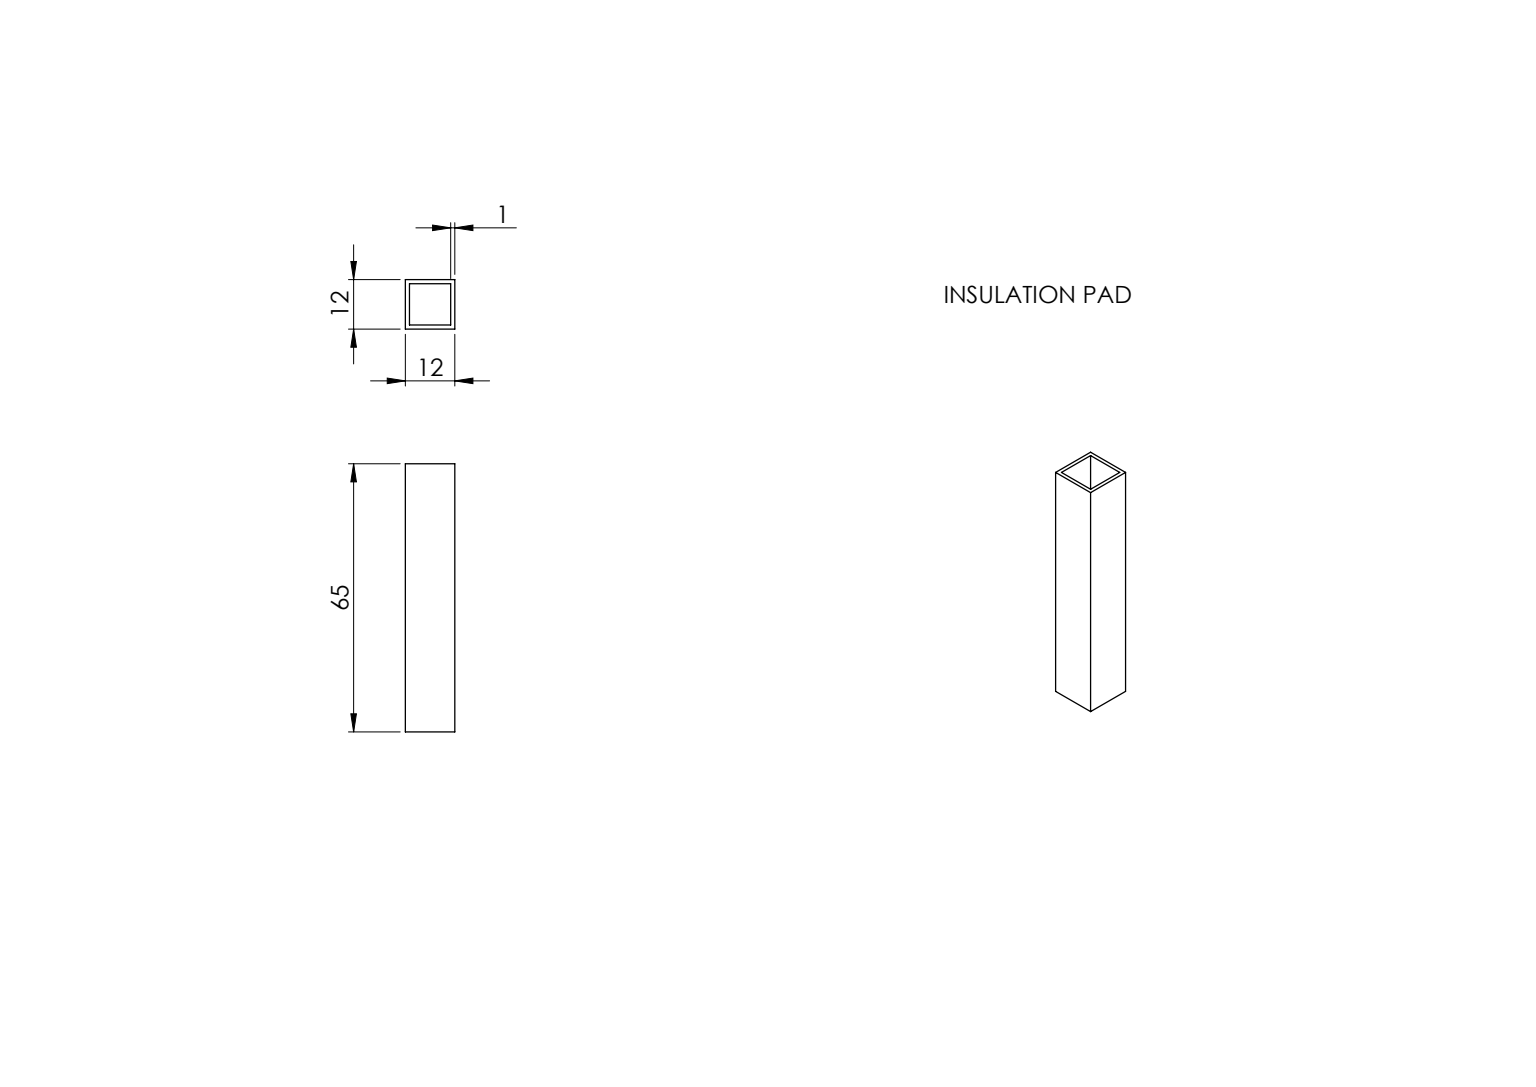
ISO-10303-21;
HEADER;
FILE_DESCRIPTION (('STEP AP214'),
    '1' );
FILE_NAME ('Insulation Pad.step',
    '2026-10-24T04:45:50',
    ( '' ),
    ( '' ),
    'SwSTEP 2.0',
    'SolidWorks 2026',
    '' );
FILE_SCHEMA (( 'AUTOMOTIVE_DESIGN' ));
ENDSEC;

DATA;
#9=LINE ( 'NONE', #3109, #1942 ) ;
#10=ORIENTED_EDGE ( 'NONE', *, *, #1397, .T. ) ;
#12=FILL_AREA_STYLE_COLOUR ( '', #2947 ) ;
#16=EDGE_CURVE ( 'NONE', #2394, #756, #2740, .T. ) ;
#20=CARTESIAN_POINT ( 'NONE',  ( -40.00000000000000000, 136.9705627484771355, -4.999999999999995559 ) ) ;
#23=CARTESIAN_POINT ( 'NONE',  ( -49.99999999999999289, 136.9705627484771355, -4.999999999999995559 ) ) ;
#29=LINE ( 'NONE', #1074, #3100 ) ;
#37=PLANE ( 'NONE',  #2989 ) ;
#53=CARTESIAN_POINT ( 'NONE',  ( -51.00000000000000000, 52.00000000000000711, -5.999999999999995559 ) ) ;
#60=EDGE_CURVE ( 'NONE', #1345, #1406, #445, .T. ) ;
#63=SHAPE_REPRESENTATION_RELATIONSHIP ( 'NONE' , 'NONE' ,  #2804, #1506 ) ;
#67=LINE ( 'NONE', #1330, #689 ) ;
#83=CARTESIAN_POINT ( 'NONE',  ( -51.00000000000000711, 136.9705627484771355, 6.000000000000004441 ) ) ;
#84=VERTEX_POINT ( 'NONE', #2233 ) ;
#102=EDGE_LOOP ( 'NONE', ( #2901, #2851, #579, #3094 ) ) ;
#105=PLANE ( 'NONE',  #1846 ) ;
#108=VERTEX_POINT ( 'NONE', #676 ) ;
#120=ORIENTED_EDGE ( 'NONE', *, *, #698, .T. ) ;
#127=ORIENTED_EDGE ( 'NONE', *, *, #1397, .F. ) ;
#136=CARTESIAN_POINT ( 'NONE',  ( 0.000000000000000000, 117.0000000000000000, 0.000000000000000000 ) ) ;
#152=VECTOR ( 'NONE', #2701, 1000.000000000000000 ) ;
#156=DIRECTION ( 'NONE',  ( 1.000000000000000000, 0.000000000000000000, -0.000000000000000000 ) ) ;
#161=MECHANICAL_DESIGN_GEOMETRIC_PRESENTATION_REPRESENTATION('',(#2503),#1797);
#164=VECTOR ( 'NONE', #3281, 1000.000000000000000 ) ;
#196=CARTESIAN_POINT ( 'NONE',  ( -51.00000000000000000, 136.9705627484771355, -5.999999999999995559 ) ) ;
#215=CARTESIAN_POINT ( 'NONE',  ( -40.00000000000000000, 52.00000000000000711, -4.999999999999995559 ) ) ;
#237=EDGE_LOOP ( 'NONE', ( #1273, #3223, #1162, #2040 ) ) ;
#241=EDGE_CURVE ( 'NONE', #1406, #684, #9, .T. ) ;
#253=CARTESIAN_POINT ( 'NONE',  ( -40.00000000000000000, 52.00000000000000711, 5.000000000000004441 ) ) ;
#265=DIRECTION ( 'NONE',  ( 0.000000000000000000, 0.000000000000000000, -1.000000000000000000 ) ) ;
#278=ORIENTED_EDGE ( 'NONE', *, *, #1945, .T. ) ;
#280=DIRECTION ( 'NONE',  ( 0.000000000000000000, 0.000000000000000000, -1.000000000000000000 ) ) ;
#305=LINE ( 'NONE', #901, #2667 ) ;
#309=VERTEX_POINT ( 'NONE', #1378 ) ;
#339=LINE ( 'NONE', #83, #1798 ) ;
#357=FACE_BOUND ( 'NONE', #1452, .T. ) ;
#380=DIRECTION ( 'NONE',  ( 0.000000000000000000, -0.000000000000000000, 1.000000000000000000 ) ) ;
#394=DIRECTION ( 'NONE',  ( 0.000000000000000000, 0.000000000000000000, 1.000000000000000000 ) ) ;
#406=CARTESIAN_POINT ( 'NONE',  ( -51.00000000000000000, 136.9705627484771355, -4.999999999999996447 ) ) ;
#409=EDGE_CURVE ( 'NONE', #2129, #108, #67, .T. ) ;
#412=PLANE ( 'NONE',  #1407 ) ;
#418=LINE ( 'NONE', #2471, #152 ) ;
#419=CARTESIAN_POINT ( 'NONE',  ( -50.00000000000000000, 117.0000000000000000, 5.000000000000004441 ) ) ;
#442=PLANE ( 'NONE',  #2112 ) ;
#445=LINE ( 'NONE', #3298, #1076 ) ;
#451=EDGE_LOOP ( 'NONE', ( #1435, #993, #1013, #2138 ) ) ;
#459=EDGE_CURVE ( 'NONE', #756, #1406, #418, .T. ) ;
#475=DIRECTION ( 'NONE',  ( 0.000000000000000000, -1.000000000000000000, 0.000000000000000000 ) ) ;
#490=CARTESIAN_POINT ( 'NONE',  ( -39.00000000000000000, 52.00000000000000711, -5.999999999999995559 ) ) ;
#505=SURFACE_SIDE_STYLE ('',( #2583 ) ) ;
#509=LINE ( 'NONE', #2809, #1520 ) ;
#540=VECTOR ( 'NONE', #639, 1000.000000000000000 ) ;
#568=ORIENTED_EDGE ( 'NONE', *, *, #3327, .T. ) ;
#578=PLANE ( 'NONE',  #2006 ) ;
#579=ORIENTED_EDGE ( 'NONE', *, *, #3144, .T. ) ;
#612=DIRECTION ( 'NONE',  ( 0.000000000000000000, 0.000000000000000000, 1.000000000000000000 ) ) ;
#625=VERTEX_POINT ( 'NONE', #215 ) ;
#627=CARTESIAN_POINT ( 'NONE',  ( -40.00000000000000000, 136.9705627484771355, -5.999999999999995559 ) ) ;
#632=ORIENTED_EDGE ( 'NONE', *, *, #2958, .F. ) ;
#634=LINE ( 'NONE', #948, #2276 ) ;
#639=DIRECTION ( 'NONE',  ( 1.000000000000000000, 0.000000000000000000, 0.000000000000000000 ) ) ;
#641=AXIS2_PLACEMENT_3D ( 'NONE', #1222, #3272, #3009 ) ;
#647=DIRECTION ( 'NONE',  ( -0.000000000000000000, -1.000000000000000000, -0.000000000000000000 ) ) ;
#649=VECTOR ( 'NONE', #3280, 1000.000000000000000 ) ;
#664=CARTESIAN_POINT ( 'NONE',  ( -49.99999999999999289, 136.9705627484771355, -4.999999999999995559 ) ) ;
#676=CARTESIAN_POINT ( 'NONE',  ( -40.00000000000000000, 117.0000000000000000, 5.000000000000004441 ) ) ;
#684=VERTEX_POINT ( 'NONE', #490 ) ;
#689=VECTOR ( 'NONE', #1588, 1000.000000000000000 ) ;
#698=EDGE_CURVE ( 'NONE', #2833, #625, #1646, .T. ) ;
#705=ORIENTED_EDGE ( 'NONE', *, *, #2348, .T. ) ;
#713=CARTESIAN_POINT ( 'NONE',  ( -50.00000000000000000, 117.0000000000000000, 5.000000000000004441 ) ) ;
#716=DIRECTION ( 'NONE',  ( -0.000000000000000000, -1.000000000000000000, -0.000000000000000000 ) ) ;
#718=ORIENTED_EDGE ( 'NONE', *, *, #60, .T. ) ;
#726=EDGE_LOOP ( 'NONE', ( #2242, #1959, #3250, #1072 ) ) ;
#729=DIRECTION ( 'NONE',  ( -1.000000000000000000, 0.000000000000000000, 0.000000000000000000 ) ) ;
#734=FACE_OUTER_BOUND ( 'NONE', #1714, .T. ) ;
#746=CARTESIAN_POINT ( 'NONE',  ( -39.00000000000000000, 136.9705627484771355, 5.000000000000004441 ) ) ;
#747=( LENGTH_UNIT ( ) NAMED_UNIT ( * ) SI_UNIT ( .MILLI., .METRE. ) );
#756=VERTEX_POINT ( 'NONE', #1175 ) ;
#761=VECTOR ( 'NONE', #1874, 1000.000000000000000 ) ;
#780=ORIENTED_EDGE ( 'NONE', *, *, #1489, .F. ) ;
#790=CARTESIAN_POINT ( 'NONE',  ( -50.00000000000000000, 136.9705627484771355, 5.000000000000004441 ) ) ;
#833=CARTESIAN_POINT ( 'NONE',  ( -39.00000000000000000, 136.9705627484771355, -5.999999999999995559 ) ) ;
#839=ORIENTED_EDGE ( 'NONE', *, *, #241, .T. ) ;
#854=FACE_OUTER_BOUND ( 'NONE', #1573, .T. ) ;
#868=EDGE_CURVE ( 'NONE', #2623, #2345, #2510, .T. ) ;
#879=ADVANCED_FACE ( 'NONE', ( #3023 ), #2238, .T. ) ;
#901=CARTESIAN_POINT ( 'NONE',  ( -49.99999999999999289, 117.0000000000000000, -4.999999999999995559 ) ) ;
#924=CARTESIAN_POINT ( 'NONE',  ( -50.00000000000000000, 136.9705627484771355, 6.000000000000004441 ) ) ;
#943=ORIENTED_EDGE ( 'NONE', *, *, #459, .F. ) ;
#948=CARTESIAN_POINT ( 'NONE',  ( -50.00000000000000000, 136.9705627484771355, 5.000000000000004441 ) ) ;
#955=DIRECTION ( 'NONE',  ( 1.000000000000000000, 0.000000000000000000, 0.000000000000000000 ) ) ;
#960=ADVANCED_FACE ( 'NONE', ( #734 ), #412, .T. ) ;
#967=LINE ( 'NONE', #419, #649 ) ;
#985=STYLED_ITEM ( 'NONE', ( #3121 ), #1506 ) ;
#987=EDGE_LOOP ( 'NONE', ( #2562, #705, #1656, #127 ) ) ;
#993=ORIENTED_EDGE ( 'NONE', *, *, #16, .F. ) ;
#995=DIRECTION ( 'NONE',  ( 0.000000000000000000, -0.000000000000000000, 1.000000000000000000 ) ) ;
#1013=ORIENTED_EDGE ( 'NONE', *, *, #1945, .F. ) ;
#1016=EDGE_LOOP ( 'NONE', ( #943, #568, #1889, #718 ) ) ;
#1021=EDGE_CURVE ( 'NONE', #84, #309, #1844, .T. ) ;
#1043=ADVANCED_FACE ( 'NONE', ( #2321 ), #2375, .T. ) ;
#1048=ORIENTED_EDGE ( 'NONE', *, *, #3063, .F. ) ;
#1052=ADVANCED_FACE ( 'NONE', ( #1083 ), #37, .T. ) ;
#1072=ORIENTED_EDGE ( 'NONE', *, *, #1390, .F. ) ;
#1074=CARTESIAN_POINT ( 'NONE',  ( -40.00000000000000000, 52.00000000000000711, -5.999999999999995559 ) ) ;
#1076=VECTOR ( 'NONE', #955, 1000.000000000000000 ) ;
#1083=FACE_OUTER_BOUND ( 'NONE', #237, .T. ) ;
#1102=LINE ( 'NONE', #3195, #761 ) ;
#1112=( NAMED_UNIT ( * ) SI_UNIT ( $, .STERADIAN. ) SOLID_ANGLE_UNIT ( ) );
#1132=DIRECTION ( 'NONE',  ( -0.000000000000000000, -1.000000000000000000, -0.000000000000000000 ) ) ;
#1162=ORIENTED_EDGE ( 'NONE', *, *, #1845, .F. ) ;
#1175=CARTESIAN_POINT ( 'NONE',  ( -39.00000000000000000, 117.0000000000000000, 6.000000000000004441 ) ) ;
#1193=CARTESIAN_POINT ( 'NONE',  ( -40.00000000000000000, 117.0000000000000000, -5.999999999999995559 ) ) ;
#1200=DIRECTION ( 'NONE',  ( -1.000000000000000000, 0.000000000000000000, -0.000000000000000000 ) ) ;
#1221=ORIENTED_EDGE ( 'NONE', *, *, #868, .T. ) ;
#1222=CARTESIAN_POINT ( 'NONE',  ( -40.00000000000000000, 136.9705627484771355, 5.000000000000004441 ) ) ;
#1232=DIRECTION ( 'NONE',  ( 0.000000000000000000, 0.000000000000000000, -1.000000000000000000 ) ) ;
#1263=( GEOMETRIC_REPRESENTATION_CONTEXT ( 3 ) GLOBAL_UNCERTAINTY_ASSIGNED_CONTEXT ( ( #2493 ) ) GLOBAL_UNIT_ASSIGNED_CONTEXT ( ( #1560, #1854, #1112 ) ) REPRESENTATION_CONTEXT ( 'NONE', 'WORKASPACE' ) );
#1273=ORIENTED_EDGE ( 'NONE', *, *, #1950, .F. ) ;
#1292=ORIENTED_EDGE ( 'NONE', *, *, #241, .F. ) ;
#1311=EDGE_CURVE ( 'NONE', #625, #2623, #2265, .T. ) ;
#1330=CARTESIAN_POINT ( 'NONE',  ( -40.00000000000000000, 117.0000000000000000, 5.000000000000004441 ) ) ;
#1334=ORIENTED_EDGE ( 'NONE', *, *, #3070, .T. ) ;
#1341=ADVANCED_FACE ( 'NONE', ( #3314 ), #2522, .F. ) ;
#1345=VERTEX_POINT ( 'NONE', #1961 ) ;
#1370=DIRECTION ( 'NONE',  ( 0.000000000000000000, 1.000000000000000000, -0.000000000000000000 ) ) ;
#1378=CARTESIAN_POINT ( 'NONE',  ( -51.00000000000000000, 117.0000000000000000, -5.999999999999995559 ) ) ;
#1382=ORIENTED_EDGE ( 'NONE', *, *, #1311, .F. ) ;
#1389=EDGE_LOOP ( 'NONE', ( #1221, #2124, #120, #3042 ) ) ;
#1390=EDGE_CURVE ( 'NONE', #108, #2833, #3056, .T. ) ;
#1397=EDGE_CURVE ( 'NONE', #3137, #2623, #1940, .T. ) ;
#1406=VERTEX_POINT ( 'NONE', #2234 ) ;
#1407=AXIS2_PLACEMENT_3D ( 'NONE', #3287, #995, #156 ) ;
#1435=ORIENTED_EDGE ( 'NONE', *, *, #3327, .F. ) ;
#1452=EDGE_LOOP ( 'NONE', ( #1334, #2743, #2444, #3065 ) ) ;
#1460=DIRECTION ( 'NONE',  ( 6.938893903907229364E-16, 0.000000000000000000, -1.000000000000000000 ) ) ;
#1484=CARTESIAN_POINT ( 'NONE',  ( -40.00000000000000000, 52.00000000000000711, -4.999999999999995559 ) ) ;
#1489=EDGE_CURVE ( 'NONE', #3137, #2129, #509, .T. ) ;
#1506=ADVANCED_BREP_SHAPE_REPRESENTATION ( '', ( #2945, #3111 ), #2889 ) ;
#1520=VECTOR ( 'NONE', #3073, 1000.000000000000000 ) ;
#1522=EDGE_LOOP ( 'NONE', ( #632, #2728, #1292, #2496 ) ) ;
#1526=PRODUCT_DEFINITION ( 'UNKNOWN', '', #2020, #3077 ) ;
#1540=DIRECTION ( 'NONE',  ( 1.000000000000000000, -0.000000000000000000, 6.938893903907229364E-16 ) ) ;
#1552=( NAMED_UNIT ( * ) SI_UNIT ( $, .STERADIAN. ) SOLID_ANGLE_UNIT ( ) );
#1560=( LENGTH_UNIT ( ) NAMED_UNIT ( * ) SI_UNIT ( .MILLI., .METRE. ) );
#1573=EDGE_LOOP ( 'NONE', ( #2660, #278, #1578, #1896 ) ) ;
#1574=DIRECTION ( 'NONE',  ( 6.938893903907229364E-16, 0.000000000000000000, -1.000000000000000000 ) ) ;
#1578=ORIENTED_EDGE ( 'NONE', *, *, #3063, .T. ) ;
#1588=DIRECTION ( 'NONE',  ( 0.000000000000000000, 0.000000000000000000, 1.000000000000000000 ) ) ;
#1602=DIRECTION ( 'NONE',  ( 0.000000000000000000, 0.000000000000000000, 1.000000000000000000 ) ) ;
#1616=ADVANCED_FACE ( 'NONE', ( #3086 ), #2849, .F. ) ;
#1646=LINE ( 'NONE', #2175, #2002 ) ;
#1649=CARTESIAN_POINT ( 'NONE',  ( -40.00000000000000000, 117.0000000000000000, -4.999999999999995559 ) ) ;
#1656=ORIENTED_EDGE ( 'NONE', *, *, #868, .F. ) ;
#1679=ORIENTED_EDGE ( 'NONE', *, *, #16, .T. ) ;
#1682=AXIS2_PLACEMENT_3D ( 'NONE', #23, #1540, #1574 ) ;
#1693=CARTESIAN_POINT ( 'NONE',  ( -39.00000000000000000, 117.0000000000000000, 5.000000000000004441 ) ) ;
#1711=UNCERTAINTY_MEASURE_WITH_UNIT (LENGTH_MEASURE( 1.000000000000000082E-05 ), #3067, 'distance_accuracy_value', 'NONE');
#1714=EDGE_LOOP ( 'NONE', ( #780, #10, #1382, #3341 ) ) ;
#1785=CARTESIAN_POINT ( 'NONE',  ( -50.00000000000000000, 117.0000000000000000, 6.000000000000004441 ) ) ;
#1793=VECTOR ( 'NONE', #716, 1000.000000000000000 ) ;
#1796=CARTESIAN_POINT ( 'NONE',  ( -51.00000000000000000, 117.0000000000000000, -4.999999999999996447 ) ) ;
#1797=( GEOMETRIC_REPRESENTATION_CONTEXT ( 3 ) GLOBAL_UNCERTAINTY_ASSIGNED_CONTEXT ( ( #2842 ) ) GLOBAL_UNIT_ASSIGNED_CONTEXT ( ( #747, #2575, #1552 ) ) REPRESENTATION_CONTEXT ( 'NONE', 'WORKASPACE' ) );
#1798=VECTOR ( 'NONE', #1132, 1000.000000000000000 ) ;
#1815=ADVANCED_FACE ( 'NONE', ( #1973 ), #442, .F. ) ;
#1825=DIRECTION ( 'NONE',  ( 6.938893903907229364E-16, 0.000000000000000000, -1.000000000000000000 ) ) ;
#1829=( NAMED_UNIT ( * ) SI_UNIT ( $, .STERADIAN. ) SOLID_ANGLE_UNIT ( ) );
#1833=LINE ( 'NONE', #1785, #2288 ) ;
#1844=LINE ( 'NONE', #1796, #2336 ) ;
#1845=EDGE_CURVE ( 'NONE', #2345, #2833, #2245, .T. ) ;
#1846=AXIS2_PLACEMENT_3D ( 'NONE', #136, #475, #2537 ) ;
#1854=( NAMED_UNIT ( * ) PLANE_ANGLE_UNIT ( ) SI_UNIT ( $, .RADIAN. ) );
#1871=CARTESIAN_POINT ( 'NONE',  ( 0.000000000000000000, 0.000000000000000000, 0.000000000000000000 ) ) ;
#1874=DIRECTION ( 'NONE',  ( -6.938893903907228378E-16, 0.000000000000000000, 1.000000000000000000 ) ) ;
#1879=DIRECTION ( 'NONE',  ( 1.000000000000000000, 0.000000000000000000, -0.000000000000000000 ) ) ;
#1889=ORIENTED_EDGE ( 'NONE', *, *, #3125, .T. ) ;
#1896=ORIENTED_EDGE ( 'NONE', *, *, #2101, .T. ) ;
#1916=CARTESIAN_POINT ( 'NONE',  ( -49.99999999999999289, 52.00000000000000711, -4.999999999999995559 ) ) ;
#1930=PLANE ( 'NONE',  #2497 ) ;
#1940=LINE ( 'NONE', #664, #3326 ) ;
#1942=VECTOR ( 'NONE', #2794, 1000.000000000000000 ) ;
#1945=EDGE_CURVE ( 'NONE', #309, #2394, #3248, .T. ) ;
#1950=EDGE_CURVE ( 'NONE', #108, #3133, #967, .T. ) ;
#1959=ORIENTED_EDGE ( 'NONE', *, *, #2868, .T. ) ;
#1961=CARTESIAN_POINT ( 'NONE',  ( -51.00000000000000711, 52.00000000000000711, 6.000000000000004441 ) ) ;
#1967=PRODUCT_CONTEXT ( 'NONE', #2725, 'mechanical' ) ;
#1973=FACE_OUTER_BOUND ( 'NONE', #102, .T. ) ;
#2002=VECTOR ( 'NONE', #265, 1000.000000000000000 ) ;
#2006=AXIS2_PLACEMENT_3D ( 'NONE', #2957, #1370, #612 ) ;
#2020=PRODUCT_DEFINITION_FORMATION_WITH_SPECIFIED_SOURCE ( 'ANY', '', #2551, .NOT_KNOWN. ) ;
#2039=PRODUCT_DEFINITION_SHAPE ( 'NONE', 'NONE',  #1526 ) ;
#2040=ORIENTED_EDGE ( 'NONE', *, *, #2348, .F. ) ;
#2101=EDGE_CURVE ( 'NONE', #684, #3122, #29, .T. ) ;
#2105=CLOSED_SHELL ( 'NONE', ( #2661, #1815, #1341, #1616, #2638, #1043, #1052, #879, #960, #2738 ) ) ;
#2112=AXIS2_PLACEMENT_3D ( 'NONE', #406, #2979, #1460 ) ;
#2124=ORIENTED_EDGE ( 'NONE', *, *, #1845, .T. ) ;
#2129=VERTEX_POINT ( 'NONE', #1649 ) ;
#2130=MECHANICAL_DESIGN_GEOMETRIC_PRESENTATION_REPRESENTATION('',(#985),#1263);
#2138=ORIENTED_EDGE ( 'NONE', *, *, #1021, .F. ) ;
#2175=CARTESIAN_POINT ( 'NONE',  ( -40.00000000000000000, 52.00000000000000711, 5.000000000000004441 ) ) ;
#2200=DIRECTION ( 'NONE',  ( -0.000000000000000000, -1.000000000000000000, -0.000000000000000000 ) ) ;
#2210=CARTESIAN_POINT ( 'NONE',  ( -50.00000000000000000, 52.00000000000000711, 5.000000000000004441 ) ) ;
#2215=CARTESIAN_POINT ( 'NONE',  ( -40.00000000000000000, 136.9705627484771355, 5.000000000000004441 ) ) ;
#2233=CARTESIAN_POINT ( 'NONE',  ( -51.00000000000000711, 117.0000000000000000, 6.000000000000004441 ) ) ;
#2234=CARTESIAN_POINT ( 'NONE',  ( -39.00000000000000000, 52.00000000000000711, 6.000000000000004441 ) ) ;
#2238=PLANE ( 'NONE',  #641 ) ;
#2242=ORIENTED_EDGE ( 'NONE', *, *, #409, .F. ) ;
#2245=LINE ( 'NONE', #3030, #540 ) ;
#2247=CARTESIAN_POINT ( 'NONE',  ( -49.99999999999999289, 117.0000000000000000, -4.999999999999995559 ) ) ;
#2265=LINE ( 'NONE', #1484, #2281 ) ;
#2276=VECTOR ( 'NONE', #2719, 1000.000000000000000 ) ;
#2281=VECTOR ( 'NONE', #2506, 1000.000000000000000 ) ;
#2288=VECTOR ( 'NONE', #729, 1000.000000000000000 ) ;
#2296=( NAMED_UNIT ( * ) PLANE_ANGLE_UNIT ( ) SI_UNIT ( $, .RADIAN. ) );
#2321=FACE_OUTER_BOUND ( 'NONE', #987, .T. ) ;
#2326=SURFACE_STYLE_USAGE ( .BOTH. , #505 ) ;
#2336=VECTOR ( 'NONE', #1825, 1000.000000000000000 ) ;
#2345=VERTEX_POINT ( 'NONE', #2210 ) ;
#2348=EDGE_CURVE ( 'NONE', #3133, #2345, #634, .T. ) ;
#2375=PLANE ( 'NONE',  #1682 ) ;
#2384=AXIS2_PLACEMENT_3D ( 'NONE', #746, #2589, #1602 ) ;
#2394=VERTEX_POINT ( 'NONE', #3119 ) ;
#2418=LINE ( 'NONE', #833, #2556 ) ;
#2441=FACE_OUTER_BOUND ( 'NONE', #451, .T. ) ;
#2444=ORIENTED_EDGE ( 'NONE', *, *, #409, .T. ) ;
#2447=AXIS2_PLACEMENT_3D ( 'NONE', #924, #1232, #1200 ) ;
#2463=FACE_OUTER_BOUND ( 'NONE', #1522, .T. ) ;
#2471=CARTESIAN_POINT ( 'NONE',  ( -39.00000000000000000, 136.9705627484771355, 6.000000000000004441 ) ) ;
#2486=LINE ( 'NONE', #196, #164 ) ;
#2493=UNCERTAINTY_MEASURE_WITH_UNIT (LENGTH_MEASURE( 1.000000000000000082E-05 ), #1560, 'distance_accuracy_value', 'NONE');
#2496=ORIENTED_EDGE ( 'NONE', *, *, #60, .F. ) ;
#2497=AXIS2_PLACEMENT_3D ( 'NONE', #627, #380, #1879 ) ;
#2503=STYLED_ITEM('',(#3408),#2945);
#2506=DIRECTION ( 'NONE',  ( -1.000000000000000000, 0.000000000000000000, 0.000000000000000000 ) ) ;
#2510=LINE ( 'NONE', #2733, #2659 ) ;
#2522=PLANE ( 'NONE',  #2447 ) ;
#2537=DIRECTION ( 'NONE',  ( 0.000000000000000000, -0.000000000000000000, -1.000000000000000000 ) ) ;
#2551=PRODUCT ( 'Insulation Pad', 'Insulation Pad', '', ( #1967 ) ) ;
#2556=VECTOR ( 'NONE', #2200, 1000.000000000000000 ) ;
#2561=LINE ( 'NONE', #20, #2884 ) ;
#2562=ORIENTED_EDGE ( 'NONE', *, *, #3070, .F. ) ;
#2575=( NAMED_UNIT ( * ) PLANE_ANGLE_UNIT ( ) SI_UNIT ( $, .RADIAN. ) );
#2583=SURFACE_STYLE_FILL_AREA ( #2821 ) ;
#2589=DIRECTION ( 'NONE',  ( -1.000000000000000000, 0.000000000000000000, 0.000000000000000000 ) ) ;
#2612=DIRECTION ( 'NONE',  ( -0.000000000000000000, -1.000000000000000000, -0.000000000000000000 ) ) ;
#2623=VERTEX_POINT ( 'NONE', #1916 ) ;
#2638=ADVANCED_FACE ( 'NONE', ( #854 ), #1930, .F. ) ;
#2639=DIRECTION ( 'NONE',  ( 1.000000000000000000, 0.000000000000000000, 0.000000000000000000 ) ) ;
#2659=VECTOR ( 'NONE', #3062, 1000.000000000000000 ) ;
#2660=ORIENTED_EDGE ( 'NONE', *, *, #3144, .F. ) ;
#2661=ADVANCED_FACE ( 'NONE', ( #2463, #3253 ), #578, .F. ) ;
#2667=VECTOR ( 'NONE', #2982, 1000.000000000000000 ) ;
#2672=DIRECTION ( 'NONE',  ( -1.000000000000000000, 0.000000000000000000, 0.000000000000000000 ) ) ;
#2701=DIRECTION ( 'NONE',  ( -0.000000000000000000, -1.000000000000000000, -0.000000000000000000 ) ) ;
#2719=DIRECTION ( 'NONE',  ( -0.000000000000000000, -1.000000000000000000, -0.000000000000000000 ) ) ;
#2725=APPLICATION_CONTEXT ( 'automotive_design' ) ;
#2728=ORIENTED_EDGE ( 'NONE', *, *, #2101, .F. ) ;
#2733=CARTESIAN_POINT ( 'NONE',  ( -49.99999999999999289, 52.00000000000000711, -4.999999999999995559 ) ) ;
#2738=ADVANCED_FACE ( 'NONE', ( #357, #2441 ), #105, .F. ) ;
#2740=LINE ( 'NONE', #1693, #3087 ) ;
#2743=ORIENTED_EDGE ( 'NONE', *, *, #1489, .T. ) ;
#2794=DIRECTION ( 'NONE',  ( 0.000000000000000000, 0.000000000000000000, -1.000000000000000000 ) ) ;
#2804=SHAPE_REPRESENTATION ( 'Insulation Pad', ( #3111 ), #2889 ) ;
#2809=CARTESIAN_POINT ( 'NONE',  ( -40.00000000000000000, 117.0000000000000000, -4.999999999999995559 ) ) ;
#2821=FILL_AREA_STYLE ('',( #12 ) ) ;
#2833=VERTEX_POINT ( 'NONE', #253 ) ;
#2842=UNCERTAINTY_MEASURE_WITH_UNIT (LENGTH_MEASURE( 1.000000000000000082E-05 ), #747, 'distance_accuracy_value', 'NONE');
#2849=PLANE ( 'NONE',  #2384 ) ;
#2851=ORIENTED_EDGE ( 'NONE', *, *, #1021, .T. ) ;
#2868=EDGE_CURVE ( 'NONE', #2129, #625, #2561, .T. ) ;
#2872=VECTOR ( 'NONE', #3310, 1000.000000000000000 ) ;
#2884=VECTOR ( 'NONE', #2612, 1000.000000000000000 ) ;
#2889=( GEOMETRIC_REPRESENTATION_CONTEXT ( 3 ) GLOBAL_UNCERTAINTY_ASSIGNED_CONTEXT ( ( #1711 ) ) GLOBAL_UNIT_ASSIGNED_CONTEXT ( ( #3067, #2296, #1829 ) ) REPRESENTATION_CONTEXT ( 'NONE', 'WORKASPACE' ) );
#2900=APPLICATION_CONTEXT ( 'automotive_design' ) ;
#2901=ORIENTED_EDGE ( 'NONE', *, *, #3125, .F. ) ;
#2945=MANIFOLD_SOLID_BREP ( 'Extrude-Thin1', #2105 ) ;
#2947=COLOUR_RGB ( '',0.8941176470588234615, 0.8941176470588234615, 0.8941176470588234615 ) ;
#2957=CARTESIAN_POINT ( 'NONE',  ( 0.000000000000000000, 52.00000000000000711, 0.000000000000000000 ) ) ;
#2958=EDGE_CURVE ( 'NONE', #3122, #1345, #1102, .T. ) ;
#2979=DIRECTION ( 'NONE',  ( 1.000000000000000000, -0.000000000000000000, 6.938893903907229364E-16 ) ) ;
#2982=DIRECTION ( 'NONE',  ( 6.938893903907229364E-16, 0.000000000000000000, -1.000000000000000000 ) ) ;
#2989=AXIS2_PLACEMENT_3D ( 'NONE', #790, #280, #3170 ) ;
#3009=DIRECTION ( 'NONE',  ( 0.000000000000000000, 0.000000000000000000, 1.000000000000000000 ) ) ;
#3023=FACE_OUTER_BOUND ( 'NONE', #726, .T. ) ;
#3030=CARTESIAN_POINT ( 'NONE',  ( -50.00000000000000000, 52.00000000000000711, 5.000000000000004441 ) ) ;
#3042=ORIENTED_EDGE ( 'NONE', *, *, #1311, .T. ) ;
#3056=LINE ( 'NONE', #2215, #1793 ) ;
#3062=DIRECTION ( 'NONE',  ( -6.938893903907228378E-16, 0.000000000000000000, 1.000000000000000000 ) ) ;
#3063=EDGE_CURVE ( 'NONE', #2394, #684, #2418, .T. ) ;
#3065=ORIENTED_EDGE ( 'NONE', *, *, #1950, .T. ) ;
#3067=( LENGTH_UNIT ( ) NAMED_UNIT ( * ) SI_UNIT ( .MILLI., .METRE. ) );
#3070=EDGE_CURVE ( 'NONE', #3133, #3137, #305, .T. ) ;
#3073=DIRECTION ( 'NONE',  ( 1.000000000000000000, 0.000000000000000000, 0.000000000000000000 ) ) ;
#3077=PRODUCT_DEFINITION_CONTEXT ( 'detailed design', #2900, 'design' ) ;
#3086=FACE_OUTER_BOUND ( 'NONE', #3188, .T. ) ;
#3087=VECTOR ( 'NONE', #394, 1000.000000000000000 ) ;
#3094=ORIENTED_EDGE ( 'NONE', *, *, #2958, .T. ) ;
#3100=VECTOR ( 'NONE', #2672, 1000.000000000000000 ) ;
#3109=CARTESIAN_POINT ( 'NONE',  ( -39.00000000000000000, 52.00000000000000711, 5.000000000000004441 ) ) ;
#3111=AXIS2_PLACEMENT_3D ( 'NONE', #1871, #3207, #2639 ) ;
#3119=CARTESIAN_POINT ( 'NONE',  ( -39.00000000000000000, 117.0000000000000000, -5.999999999999995559 ) ) ;
#3121=PRESENTATION_STYLE_ASSIGNMENT (( #2326 ) ) ;
#3122=VERTEX_POINT ( 'NONE', #53 ) ;
#3125=EDGE_CURVE ( 'NONE', #84, #1345, #339, .T. ) ;
#3133=VERTEX_POINT ( 'NONE', #713 ) ;
#3137=VERTEX_POINT ( 'NONE', #2247 ) ;
#3144=EDGE_CURVE ( 'NONE', #309, #3122, #2486, .T. ) ;
#3170=DIRECTION ( 'NONE',  ( -1.000000000000000000, 0.000000000000000000, -0.000000000000000000 ) ) ;
#3188=EDGE_LOOP ( 'NONE', ( #1048, #1679, #3347, #839 ) ) ;
#3195=CARTESIAN_POINT ( 'NONE',  ( -51.00000000000000000, 52.00000000000000711, -4.999999999999996447 ) ) ;
#3207=DIRECTION ( 'NONE',  ( 0.000000000000000000, 0.000000000000000000, 1.000000000000000000 ) ) ;
#3223=ORIENTED_EDGE ( 'NONE', *, *, #1390, .T. ) ;
#3248=LINE ( 'NONE', #1193, #2872 ) ;
#3250=ORIENTED_EDGE ( 'NONE', *, *, #698, .F. ) ;
#3253=FACE_BOUND ( 'NONE', #1389, .T. ) ;
#3272=DIRECTION ( 'NONE',  ( -1.000000000000000000, 0.000000000000000000, 0.000000000000000000 ) ) ;
#3280=DIRECTION ( 'NONE',  ( -1.000000000000000000, 0.000000000000000000, 0.000000000000000000 ) ) ;
#3281=DIRECTION ( 'NONE',  ( -0.000000000000000000, -1.000000000000000000, -0.000000000000000000 ) ) ;
#3287=CARTESIAN_POINT ( 'NONE',  ( -40.00000000000000000, 136.9705627484771355, -4.999999999999995559 ) ) ;
#3289=SHAPE_DEFINITION_REPRESENTATION ( #2039, #2804 ) ;
#3298=CARTESIAN_POINT ( 'NONE',  ( -50.00000000000000000, 52.00000000000000711, 6.000000000000004441 ) ) ;
#3310=DIRECTION ( 'NONE',  ( 1.000000000000000000, 0.000000000000000000, 0.000000000000000000 ) ) ;
#3314=FACE_OUTER_BOUND ( 'NONE', #1016, .T. ) ;
#3326=VECTOR ( 'NONE', #647, 1000.000000000000000 ) ;
#3327=EDGE_CURVE ( 'NONE', #756, #84, #1833, .T. ) ;
#3341=ORIENTED_EDGE ( 'NONE', *, *, #2868, .F. ) ;
#3347=ORIENTED_EDGE ( 'NONE', *, *, #459, .T. ) ;
#3402=COLOUR_RGB('Sky Blue',0.24,0.69,0.87);
#3403=FILL_AREA_STYLE_COLOUR('',#3402);
#3404=FILL_AREA_STYLE('',(#3403));
#3405=SURFACE_STYLE_FILL_AREA(#3404);
#3406=SURFACE_SIDE_STYLE('',(#3405));
#3407=SURFACE_STYLE_USAGE(.BOTH.,#3406);
#3408=PRESENTATION_STYLE_ASSIGNMENT((#3407));
ENDSEC;
END-ISO-10303-21;
